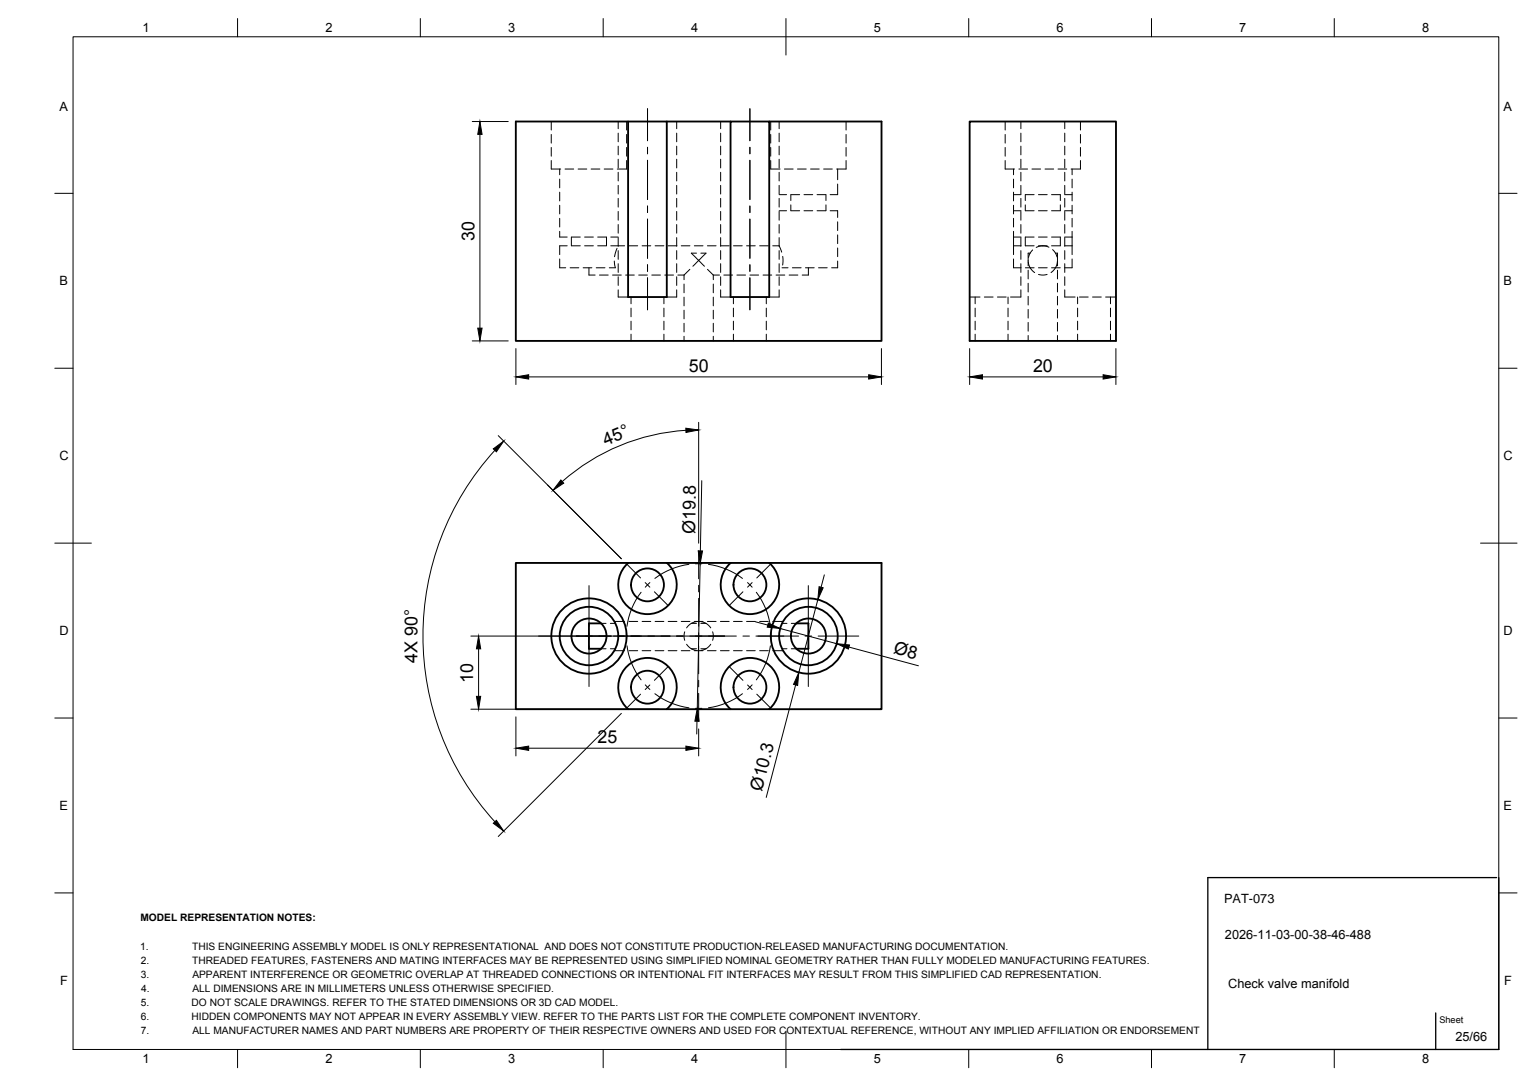
ISO-10303-21;
HEADER;
/* Generated by software containing ST-Developer
 * from STEP Tools, Inc. (www.steptools.com) 
 */

FILE_DESCRIPTION(
/* description */ ('Manual piston pump'),
/* implementation_level */ '2;1');

FILE_NAME(
/* name */ 'Check valve manifold.step',
/* time_stamp */ '2026-11-02T16:54:23-08:00',
/* author */ (''),
/* organization */ (''),
/* preprocessor_version */ 'ST-DEVELOPER v20.2',
/* originating_system */ 'Autodesk Translation Framework v15.17.0.0',
/* authorisation */ '');

FILE_SCHEMA (('AUTOMOTIVE_DESIGN { 1 0 10303 214 3 1 1 }'));
ENDSEC;

DATA;
#10=MECHANICAL_DESIGN_GEOMETRIC_PRESENTATION_REPRESENTATION('',(#725),#19043);
#13=ELLIPSE('',#10933,0.282842712474619,0.2);
#14=ELLIPSE('',#10934,0.282842712474619,0.2);
#15=ELLIPSE('',#10935,0.282842712474619,0.2);
#16=ELLIPSE('',#10936,0.282842712474619,0.2);
#17=ELLIPSE('',#10937,0.282842712474619,0.2);
#18=ELLIPSE('',#10938,0.282842712474619,0.2);
#19=ELLIPSE('',#10939,0.282842712474619,0.2);
#591=SHAPE_REPRESENTATION_RELATIONSHIP('SRR','None',#19338,#654);
#654=ADVANCED_BREP_SHAPE_REPRESENTATION('',(#795),#19005);
#725=STYLED_ITEM('',(#19661),#795);
#795=MANIFOLD_SOLID_BREP('Body1',#9511);
#966=FACE_BOUND('',#2306,.T.);
#967=FACE_BOUND('',#2309,.T.);
#968=FACE_BOUND('',#2312,.T.);
#969=FACE_BOUND('',#2315,.T.);
#970=FACE_BOUND('',#2319,.T.);
#971=FACE_BOUND('',#2320,.T.);
#972=FACE_BOUND('',#2328,.T.);
#973=FACE_BOUND('',#2331,.T.);
#974=FACE_BOUND('',#2336,.T.);
#975=FACE_BOUND('',#2340,.T.);
#976=FACE_BOUND('',#2343,.T.);
#977=FACE_BOUND('',#2348,.T.);
#978=FACE_BOUND('',#2351,.T.);
#979=FACE_BOUND('',#2360,.T.);
#980=FACE_BOUND('',#2361,.T.);
#981=FACE_BOUND('',#2362,.T.);
#982=FACE_BOUND('',#2363,.T.);
#983=FACE_BOUND('',#2364,.T.);
#1069=B_SPLINE_CURVE_WITH_KNOTS('',3,(#16509,#16510,#16511,#16512,#16513,
#16514,#16515,#16516,#16517,#16518,#16519,#16520,#16521,#16522),
 .UNSPECIFIED.,.F.,.F.,(4,2,2,2,2,2,4),(0.307512441683017,0.38428562234823,
0.461058803013443,0.538041843189738,0.615024883366033,0.692007923542328,
0.716698321761712),.UNSPECIFIED.);
#1070=B_SPLINE_CURVE_WITH_KNOTS('',3,(#16524,#16525,#16526,#16527,#16528,
#16529,#16530,#16531,#16532,#16533,#16534,#16535,#16536,#16537,#16538),
 .UNSPECIFIED.,.F.,.F.,(4,2,3,2,2,2,4),(-0.101673438395677,-0.0769830401762948,
0.,0.0769830401762949,0.15396608035259,0.230739261017803,0.307512441683017),
 .UNSPECIFIED.);
#1071=B_SPLINE_CURVE_WITH_KNOTS('',3,(#16573,#16574,#16575,#16576,#16577,
#16578,#16579,#16580,#16581,#16582,#16583,#16584,#16585,#16586),
 .UNSPECIFIED.,.F.,.F.,(4,2,2,2,2,2,4),(-0.716698321761712,-0.692007923542328,
-0.615024883366033,-0.538041843189738,-0.461058803013443,-0.38428562234823,
-0.307512441683017),.UNSPECIFIED.);
#1072=B_SPLINE_CURVE_WITH_KNOTS('',3,(#16590,#16591,#16592,#16593,#16594,
#16595,#16596,#16597,#16598,#16599,#16600,#16601,#16602,#16603,#16604),
 .UNSPECIFIED.,.F.,.F.,(4,2,2,2,3,2,4),(-0.307512441683017,-0.230739261017803,
-0.15396608035259,-0.0769830401762948,0.,0.0769830401762949,0.101673438395681),
 .UNSPECIFIED.);
#1202=CYLINDRICAL_SURFACE('',#10867,0.4);
#1203=CYLINDRICAL_SURFACE('',#10872,0.4);
#1204=CYLINDRICAL_SURFACE('',#10877,0.4);
#1205=CYLINDRICAL_SURFACE('',#10882,0.4);
#1206=CYLINDRICAL_SURFACE('',#10889,0.225);
#1207=CYLINDRICAL_SURFACE('',#10891,0.225);
#1208=CYLINDRICAL_SURFACE('',#10893,0.225);
#1209=CYLINDRICAL_SURFACE('',#10895,0.225);
#1210=CYLINDRICAL_SURFACE('',#10897,0.515);
#1211=CYLINDRICAL_SURFACE('',#10901,0.4);
#1212=CYLINDRICAL_SURFACE('',#10905,0.24);
#1213=CYLINDRICAL_SURFACE('',#10909,0.4);
#1214=CYLINDRICAL_SURFACE('',#10914,0.515);
#1215=CYLINDRICAL_SURFACE('',#10918,0.4);
#1216=CYLINDRICAL_SURFACE('',#10922,0.24);
#1217=CYLINDRICAL_SURFACE('',#10927,0.4);
#1218=CYLINDRICAL_SURFACE('',#10932,0.2);
#1219=CYLINDRICAL_SURFACE('',#10944,0.2);
#1220=CYLINDRICAL_SURFACE('',#10945,0.2);
#1221=CYLINDRICAL_SURFACE('',#10946,0.2);
#1591=FACE_OUTER_BOUND('',#2305,.T.);
#1592=FACE_OUTER_BOUND('',#2307,.T.);
#1593=FACE_OUTER_BOUND('',#2308,.T.);
#1594=FACE_OUTER_BOUND('',#2310,.T.);
#1595=FACE_OUTER_BOUND('',#2311,.T.);
#1596=FACE_OUTER_BOUND('',#2313,.T.);
#1597=FACE_OUTER_BOUND('',#2314,.T.);
#1598=FACE_OUTER_BOUND('',#2316,.T.);
#1599=FACE_OUTER_BOUND('',#2317,.T.);
#1600=FACE_OUTER_BOUND('',#2318,.T.);
#1601=FACE_OUTER_BOUND('',#2321,.T.);
#1602=FACE_OUTER_BOUND('',#2322,.T.);
#1603=FACE_OUTER_BOUND('',#2323,.T.);
#1604=FACE_OUTER_BOUND('',#2324,.T.);
#1605=FACE_OUTER_BOUND('',#2325,.T.);
#1606=FACE_OUTER_BOUND('',#2326,.T.);
#1607=FACE_OUTER_BOUND('',#2327,.T.);
#1608=FACE_OUTER_BOUND('',#2329,.T.);
#1609=FACE_OUTER_BOUND('',#2330,.T.);
#1610=FACE_OUTER_BOUND('',#2332,.T.);
#1611=FACE_OUTER_BOUND('',#2333,.T.);
#1612=FACE_OUTER_BOUND('',#2334,.T.);
#1613=FACE_OUTER_BOUND('',#2335,.T.);
#1614=FACE_OUTER_BOUND('',#2337,.T.);
#1615=FACE_OUTER_BOUND('',#2338,.T.);
#1616=FACE_OUTER_BOUND('',#2339,.T.);
#1617=FACE_OUTER_BOUND('',#2341,.T.);
#1618=FACE_OUTER_BOUND('',#2342,.T.);
#1619=FACE_OUTER_BOUND('',#2344,.T.);
#1620=FACE_OUTER_BOUND('',#2345,.T.);
#1621=FACE_OUTER_BOUND('',#2346,.T.);
#1622=FACE_OUTER_BOUND('',#2347,.T.);
#1623=FACE_OUTER_BOUND('',#2349,.T.);
#1624=FACE_OUTER_BOUND('',#2350,.T.);
#1625=FACE_OUTER_BOUND('',#2352,.T.);
#1626=FACE_OUTER_BOUND('',#2353,.T.);
#1627=FACE_OUTER_BOUND('',#2354,.T.);
#1628=FACE_OUTER_BOUND('',#2355,.T.);
#1629=FACE_OUTER_BOUND('',#2356,.T.);
#1630=FACE_OUTER_BOUND('',#2357,.T.);
#1631=FACE_OUTER_BOUND('',#2358,.T.);
#1632=FACE_OUTER_BOUND('',#2359,.T.);
#2305=EDGE_LOOP('',(#7503,#7504));
#2306=EDGE_LOOP('',(#7505));
#2307=EDGE_LOOP('',(#7506,#7507,#7508,#7509));
#2308=EDGE_LOOP('',(#7510,#7511));
#2309=EDGE_LOOP('',(#7512));
#2310=EDGE_LOOP('',(#7513,#7514,#7515,#7516));
#2311=EDGE_LOOP('',(#7517,#7518));
#2312=EDGE_LOOP('',(#7519));
#2313=EDGE_LOOP('',(#7520,#7521,#7522,#7523));
#2314=EDGE_LOOP('',(#7524,#7525));
#2315=EDGE_LOOP('',(#7526));
#2316=EDGE_LOOP('',(#7527,#7528,#7529,#7530));
#2317=EDGE_LOOP('',(#7531,#7532,#7533,#7534,#7535,#7536,#7537,#7538,#7539,
#7540,#7541,#7542));
#2318=EDGE_LOOP('',(#7543,#7544,#7545,#7546,#7547,#7548,#7549,#7550,#7551,
#7552,#7553,#7554));
#2319=EDGE_LOOP('',(#7555));
#2320=EDGE_LOOP('',(#7556));
#2321=EDGE_LOOP('',(#7557,#7558,#7559,#7560,#7561,#7562,#7563,#7564,#7565,
#7566,#7567,#7568));
#2322=EDGE_LOOP('',(#7569,#7570,#7571,#7572));
#2323=EDGE_LOOP('',(#7573,#7574,#7575,#7576));
#2324=EDGE_LOOP('',(#7577,#7578,#7579,#7580));
#2325=EDGE_LOOP('',(#7581,#7582,#7583,#7584));
#2326=EDGE_LOOP('',(#7585,#7586,#7587,#7588));
#2327=EDGE_LOOP('',(#7589));
#2328=EDGE_LOOP('',(#7590));
#2329=EDGE_LOOP('',(#7591,#7592,#7593,#7594));
#2330=EDGE_LOOP('',(#7595));
#2331=EDGE_LOOP('',(#7596));
#2332=EDGE_LOOP('',(#7597,#7598,#7599,#7600));
#2333=EDGE_LOOP('',(#7601,#7602,#7603,#7604));
#2334=EDGE_LOOP('',(#7605,#7606,#7607,#7608));
#2335=EDGE_LOOP('',(#7609));
#2336=EDGE_LOOP('',(#7610));
#2337=EDGE_LOOP('',(#7611,#7612));
#2338=EDGE_LOOP('',(#7613,#7614,#7615,#7616));
#2339=EDGE_LOOP('',(#7617));
#2340=EDGE_LOOP('',(#7618));
#2341=EDGE_LOOP('',(#7619,#7620,#7621,#7622));
#2342=EDGE_LOOP('',(#7623));
#2343=EDGE_LOOP('',(#7624));
#2344=EDGE_LOOP('',(#7625,#7626,#7627,#7628));
#2345=EDGE_LOOP('',(#7629,#7630,#7631,#7632,#7633));
#2346=EDGE_LOOP('',(#7634,#7635,#7636,#7637,#7638,#7639,#7640));
#2347=EDGE_LOOP('',(#7641));
#2348=EDGE_LOOP('',(#7642));
#2349=EDGE_LOOP('',(#7643,#7644));
#2350=EDGE_LOOP('',(#7645,#7646,#7647,#7648,#7649,#7650,#7651,#7652,#7653,
#7654,#7655,#7656));
#2351=EDGE_LOOP('',(#7657,#7658,#7659,#7660,#7661,#7662,#7663,#7664,#7665));
#2352=EDGE_LOOP('',(#7666,#7667));
#2353=EDGE_LOOP('',(#7668,#7669));
#2354=EDGE_LOOP('',(#7670,#7671,#7672));
#2355=EDGE_LOOP('',(#7673,#7674,#7675));
#2356=EDGE_LOOP('',(#7676,#7677,#7678,#7679,#7680,#7681));
#2357=EDGE_LOOP('',(#7682,#7683,#7684,#7685));
#2358=EDGE_LOOP('',(#7686,#7687,#7688,#7689));
#2359=EDGE_LOOP('',(#7690,#7691,#7692,#7693));
#2360=EDGE_LOOP('',(#7694));
#2361=EDGE_LOOP('',(#7695));
#2362=EDGE_LOOP('',(#7696));
#2363=EDGE_LOOP('',(#7697));
#2364=EDGE_LOOP('',(#7698));
#2947=CIRCLE('',#10865,0.4);
#2948=CIRCLE('',#10866,0.225);
#2949=CIRCLE('',#10868,0.4);
#2950=CIRCLE('',#10870,0.4);
#2951=CIRCLE('',#10871,0.225);
#2952=CIRCLE('',#10873,0.4);
#2953=CIRCLE('',#10875,0.4);
#2954=CIRCLE('',#10876,0.225);
#2955=CIRCLE('',#10878,0.4);
#2956=CIRCLE('',#10880,0.4);
#2957=CIRCLE('',#10881,0.225);
#2958=CIRCLE('',#10883,0.4);
#2959=CIRCLE('',#10886,0.515);
#2960=CIRCLE('',#10887,0.515);
#2961=CIRCLE('',#10890,0.225);
#2962=CIRCLE('',#10892,0.225);
#2963=CIRCLE('',#10894,0.225);
#2964=CIRCLE('',#10896,0.225);
#2965=CIRCLE('',#10898,0.515);
#2966=CIRCLE('',#10900,0.4);
#2967=CIRCLE('',#10902,0.4);
#2968=CIRCLE('',#10904,0.24);
#2969=CIRCLE('',#10906,0.24);
#2970=CIRCLE('',#10908,0.4);
#2971=CIRCLE('',#10910,0.4);
#2972=CIRCLE('',#10913,0.2);
#2973=CIRCLE('',#10915,0.515);
#2974=CIRCLE('',#10917,0.4);
#2975=CIRCLE('',#10919,0.4);
#2976=CIRCLE('',#10921,0.24);
#2977=CIRCLE('',#10923,0.24);
#2978=CIRCLE('',#10925,0.4);
#2979=CIRCLE('',#10926,0.4);
#2980=CIRCLE('',#10928,0.4);
#2981=CIRCLE('',#10931,0.2);
#2982=CIRCLE('',#10941,0.2);
#2983=CIRCLE('',#10943,0.2);
#2984=CIRCLE('',#10947,0.2);
#3445=LINE('',#16386,#4049);
#3446=LINE('',#16392,#4050);
#3447=LINE('',#16395,#4051);
#3448=LINE('',#16399,#4052);
#3449=LINE('',#16405,#4053);
#3450=LINE('',#16408,#4054);
#3451=LINE('',#16412,#4055);
#3452=LINE('',#16418,#4056);
#3453=LINE('',#16421,#4057);
#3454=LINE('',#16425,#4058);
#3455=LINE('',#16431,#4059);
#3456=LINE('',#16434,#4060);
#3457=LINE('',#16436,#4061);
#3458=LINE('',#16438,#4062);
#3459=LINE('',#16440,#4063);
#3460=LINE('',#16442,#4064);
#3461=LINE('',#16444,#4065);
#3462=LINE('',#16445,#4066);
#3463=LINE('',#16448,#4067);
#3464=LINE('',#16449,#4068);
#3465=LINE('',#16450,#4069);
#3466=LINE('',#16452,#4070);
#3467=LINE('',#16453,#4071);
#3468=LINE('',#16460,#4072);
#3469=LINE('',#16462,#4073);
#3470=LINE('',#16463,#4074);
#3471=LINE('',#16467,#4075);
#3472=LINE('',#16471,#4076);
#3473=LINE('',#16475,#4077);
#3474=LINE('',#16479,#4078);
#3475=LINE('',#16483,#4079);
#3476=LINE('',#16490,#4080);
#3477=LINE('',#16497,#4081);
#3478=LINE('',#16501,#4082);
#3479=LINE('',#16505,#4083);
#3480=LINE('',#16506,#4084);
#3481=LINE('',#16545,#4085);
#3482=LINE('',#16552,#4086);
#3483=LINE('',#16559,#4087);
#3484=LINE('',#16563,#4088);
#3485=LINE('',#16569,#4089);
#3486=LINE('',#16570,#4090);
#3487=LINE('',#16588,#4091);
#3488=LINE('',#16609,#4092);
#3489=LINE('',#16616,#4093);
#3490=LINE('',#16623,#4094);
#3491=LINE('',#16635,#4095);
#3492=LINE('',#16637,#4096);
#3493=LINE('',#16639,#4097);
#4049=VECTOR('',#13037,1.);
#4050=VECTOR('',#13044,1.);
#4051=VECTOR('',#13047,1.);
#4052=VECTOR('',#13050,1.);
#4053=VECTOR('',#13057,1.);
#4054=VECTOR('',#13060,1.);
#4055=VECTOR('',#13063,1.);
#4056=VECTOR('',#13070,1.);
#4057=VECTOR('',#13073,1.);
#4058=VECTOR('',#13076,1.);
#4059=VECTOR('',#13083,1.);
#4060=VECTOR('',#13086,1.);
#4061=VECTOR('',#13089,1.);
#4062=VECTOR('',#13090,1.);
#4063=VECTOR('',#13091,1.);
#4064=VECTOR('',#13092,1.);
#4065=VECTOR('',#13093,1.);
#4066=VECTOR('',#13094,1.);
#4067=VECTOR('',#13097,1.);
#4068=VECTOR('',#13098,1.);
#4069=VECTOR('',#13099,1.);
#4070=VECTOR('',#13100,1.);
#4071=VECTOR('',#13101,1.);
#4072=VECTOR('',#13108,1.);
#4073=VECTOR('',#13109,1.);
#4074=VECTOR('',#13110,1.);
#4075=VECTOR('',#13115,0.225);
#4076=VECTOR('',#13120,0.225);
#4077=VECTOR('',#13125,0.225);
#4078=VECTOR('',#13130,0.225);
#4079=VECTOR('',#13135,0.515);
#4080=VECTOR('',#13144,0.4);
#4081=VECTOR('',#13153,0.24);
#4082=VECTOR('',#13156,1.);
#4083=VECTOR('',#13159,1.);
#4084=VECTOR('',#13160,1.);
#4085=VECTOR('',#13175,0.515);
#4086=VECTOR('',#13184,0.4);
#4087=VECTOR('',#13193,0.24);
#4088=VECTOR('',#13196,1.);
#4089=VECTOR('',#13201,1.);
#4090=VECTOR('',#13202,1.);
#4091=VECTOR('',#13205,0.4);
#4092=VECTOR('',#13216,0.2);
#4093=VECTOR('',#13221,1.);
#4094=VECTOR('',#13228,1.);
#4095=VECTOR('',#13249,0.2);
#4096=VECTOR('',#13252,1.);
#4097=VECTOR('',#13255,1.);
#4770=VERTEX_POINT('',#16384);
#4771=VERTEX_POINT('',#16385);
#4772=VERTEX_POINT('',#16388);
#4773=VERTEX_POINT('',#16391);
#4774=VERTEX_POINT('',#16393);
#4775=VERTEX_POINT('',#16397);
#4776=VERTEX_POINT('',#16398);
#4777=VERTEX_POINT('',#16401);
#4778=VERTEX_POINT('',#16404);
#4779=VERTEX_POINT('',#16406);
#4780=VERTEX_POINT('',#16410);
#4781=VERTEX_POINT('',#16411);
#4782=VERTEX_POINT('',#16414);
#4783=VERTEX_POINT('',#16417);
#4784=VERTEX_POINT('',#16419);
#4785=VERTEX_POINT('',#16423);
#4786=VERTEX_POINT('',#16424);
#4787=VERTEX_POINT('',#16427);
#4788=VERTEX_POINT('',#16430);
#4789=VERTEX_POINT('',#16432);
#4790=VERTEX_POINT('',#16437);
#4791=VERTEX_POINT('',#16439);
#4792=VERTEX_POINT('',#16441);
#4793=VERTEX_POINT('',#16443);
#4794=VERTEX_POINT('',#16447);
#4795=VERTEX_POINT('',#16451);
#4796=VERTEX_POINT('',#16454);
#4797=VERTEX_POINT('',#16456);
#4798=VERTEX_POINT('',#16459);
#4799=VERTEX_POINT('',#16461);
#4800=VERTEX_POINT('',#16465);
#4801=VERTEX_POINT('',#16469);
#4802=VERTEX_POINT('',#16473);
#4803=VERTEX_POINT('',#16477);
#4804=VERTEX_POINT('',#16481);
#4805=VERTEX_POINT('',#16485);
#4806=VERTEX_POINT('',#16488);
#4807=VERTEX_POINT('',#16492);
#4808=VERTEX_POINT('',#16495);
#4809=VERTEX_POINT('',#16499);
#4810=VERTEX_POINT('',#16500);
#4811=VERTEX_POINT('',#16502);
#4812=VERTEX_POINT('',#16504);
#4813=VERTEX_POINT('',#16508);
#4814=VERTEX_POINT('',#16543);
#4815=VERTEX_POINT('',#16547);
#4816=VERTEX_POINT('',#16550);
#4817=VERTEX_POINT('',#16554);
#4818=VERTEX_POINT('',#16557);
#4819=VERTEX_POINT('',#16561);
#4820=VERTEX_POINT('',#16562);
#4821=VERTEX_POINT('',#16564);
#4822=VERTEX_POINT('',#16566);
#4823=VERTEX_POINT('',#16568);
#4824=VERTEX_POINT('',#16572);
#4825=VERTEX_POINT('',#16587);
#4826=VERTEX_POINT('',#16610);
#4827=VERTEX_POINT('',#16611);
#4828=VERTEX_POINT('',#16613);
#4829=VERTEX_POINT('',#16615);
#4830=VERTEX_POINT('',#16618);
#4831=VERTEX_POINT('',#16620);
#4832=VERTEX_POINT('',#16622);
#4833=VERTEX_POINT('',#16633);
#5738=EDGE_CURVE('',#4770,#4771,#3445,.T.);
#5739=EDGE_CURVE('',#4770,#4771,#2947,.T.);
#5740=EDGE_CURVE('',#4772,#4772,#2948,.T.);
#5741=EDGE_CURVE('',#4773,#4770,#3446,.T.);
#5742=EDGE_CURVE('',#4774,#4773,#2949,.T.);
#5743=EDGE_CURVE('',#4771,#4774,#3447,.T.);
#5744=EDGE_CURVE('',#4775,#4776,#3448,.T.);
#5745=EDGE_CURVE('',#4775,#4776,#2950,.T.);
#5746=EDGE_CURVE('',#4777,#4777,#2951,.T.);
#5747=EDGE_CURVE('',#4778,#4775,#3449,.T.);
#5748=EDGE_CURVE('',#4779,#4778,#2952,.T.);
#5749=EDGE_CURVE('',#4776,#4779,#3450,.T.);
#5750=EDGE_CURVE('',#4780,#4781,#3451,.T.);
#5751=EDGE_CURVE('',#4780,#4781,#2953,.T.);
#5752=EDGE_CURVE('',#4782,#4782,#2954,.T.);
#5753=EDGE_CURVE('',#4783,#4780,#3452,.T.);
#5754=EDGE_CURVE('',#4784,#4783,#2955,.T.);
#5755=EDGE_CURVE('',#4781,#4784,#3453,.T.);
#5756=EDGE_CURVE('',#4785,#4786,#3454,.T.);
#5757=EDGE_CURVE('',#4785,#4786,#2956,.T.);
#5758=EDGE_CURVE('',#4787,#4787,#2957,.T.);
#5759=EDGE_CURVE('',#4788,#4785,#3455,.T.);
#5760=EDGE_CURVE('',#4789,#4788,#2958,.T.);
#5761=EDGE_CURVE('',#4786,#4789,#3456,.T.);
#5762=EDGE_CURVE('',#4783,#4774,#3457,.T.);
#5763=EDGE_CURVE('',#4790,#4784,#3458,.T.);
#5764=EDGE_CURVE('',#4791,#4790,#3459,.T.);
#5765=EDGE_CURVE('',#4791,#4792,#3460,.T.);
#5766=EDGE_CURVE('',#4792,#4793,#3461,.T.);
#5767=EDGE_CURVE('',#4773,#4793,#3462,.T.);
#5768=EDGE_CURVE('',#4793,#4794,#3463,.T.);
#5769=EDGE_CURVE('',#4794,#4789,#3464,.T.);
#5770=EDGE_CURVE('',#4788,#4779,#3465,.T.);
#5771=EDGE_CURVE('',#4778,#4795,#3466,.T.);
#5772=EDGE_CURVE('',#4795,#4790,#3467,.T.);
#5773=EDGE_CURVE('',#4796,#4796,#2959,.T.);
#5774=EDGE_CURVE('',#4797,#4797,#2960,.T.);
#5775=EDGE_CURVE('',#4798,#4794,#3468,.T.);
#5776=EDGE_CURVE('',#4798,#4799,#3469,.T.);
#5777=EDGE_CURVE('',#4799,#4795,#3470,.T.);
#5778=EDGE_CURVE('',#4800,#4800,#2961,.T.);
#5779=EDGE_CURVE('',#4800,#4772,#3471,.T.);
#5780=EDGE_CURVE('',#4801,#4801,#2962,.T.);
#5781=EDGE_CURVE('',#4801,#4777,#3472,.T.);
#5782=EDGE_CURVE('',#4802,#4802,#2963,.T.);
#5783=EDGE_CURVE('',#4802,#4782,#3473,.T.);
#5784=EDGE_CURVE('',#4803,#4803,#2964,.T.);
#5785=EDGE_CURVE('',#4803,#4787,#3474,.T.);
#5786=EDGE_CURVE('',#4804,#4804,#2965,.T.);
#5787=EDGE_CURVE('',#4804,#4796,#3475,.T.);
#5788=EDGE_CURVE('',#4805,#4805,#2966,.T.);
#5789=EDGE_CURVE('',#4806,#4806,#2967,.T.);
#5790=EDGE_CURVE('',#4806,#4805,#3476,.T.);
#5791=EDGE_CURVE('',#4807,#4807,#2968,.T.);
#5792=EDGE_CURVE('',#4808,#4808,#2969,.T.);
#5793=EDGE_CURVE('',#4808,#4807,#3477,.T.);
#5794=EDGE_CURVE('',#4809,#4810,#3478,.T.);
#5795=EDGE_CURVE('',#4809,#4811,#2970,.T.);
#5796=EDGE_CURVE('',#4812,#4811,#3479,.T.);
#5797=EDGE_CURVE('',#4810,#4812,#3480,.T.);
#5798=EDGE_CURVE('',#4813,#4809,#1069,.T.);
#5799=EDGE_CURVE('',#4813,#4813,#2971,.T.);
#5800=EDGE_CURVE('',#4811,#4813,#1070,.T.);
#5801=EDGE_CURVE('',#4810,#4812,#2972,.T.);
#5802=EDGE_CURVE('',#4814,#4814,#2973,.T.);
#5803=EDGE_CURVE('',#4814,#4797,#3481,.T.);
#5804=EDGE_CURVE('',#4815,#4815,#2974,.T.);
#5805=EDGE_CURVE('',#4816,#4816,#2975,.T.);
#5806=EDGE_CURVE('',#4816,#4815,#3482,.T.);
#5807=EDGE_CURVE('',#4817,#4817,#2976,.T.);
#5808=EDGE_CURVE('',#4818,#4818,#2977,.T.);
#5809=EDGE_CURVE('',#4818,#4817,#3483,.T.);
#5810=EDGE_CURVE('',#4819,#4820,#3484,.T.);
#5811=EDGE_CURVE('',#4819,#4821,#2978,.T.);
#5812=EDGE_CURVE('',#4821,#4822,#2979,.T.);
#5813=EDGE_CURVE('',#4823,#4822,#3485,.T.);
#5814=EDGE_CURVE('',#4820,#4823,#3486,.T.);
#5815=EDGE_CURVE('',#4822,#4824,#1071,.T.);
#5816=EDGE_CURVE('',#4821,#4825,#3487,.T.);
#5817=EDGE_CURVE('',#4825,#4825,#2980,.T.);
#5818=EDGE_CURVE('',#4824,#4819,#1072,.T.);
#5819=EDGE_CURVE('',#4823,#4820,#2981,.T.);
#5820=EDGE_CURVE('',#4824,#4813,#3488,.T.);
#5821=EDGE_CURVE('',#4826,#4827,#13,.T.);
#5822=EDGE_CURVE('',#4828,#4826,#14,.T.);
#5823=EDGE_CURVE('',#4829,#4828,#3489,.T.);
#5824=EDGE_CURVE('',#4826,#4829,#15,.T.);
#5825=EDGE_CURVE('',#4830,#4826,#16,.T.);
#5826=EDGE_CURVE('',#4831,#4830,#17,.T.);
#5827=EDGE_CURVE('',#4832,#4831,#3490,.T.);
#5828=EDGE_CURVE('',#4830,#4832,#18,.T.);
#5829=EDGE_CURVE('',#4827,#4830,#19,.T.);
#5830=EDGE_CURVE('',#4829,#4828,#2982,.T.);
#5831=EDGE_CURVE('',#4832,#4831,#2983,.T.);
#5832=EDGE_CURVE('',#4833,#4833,#2984,.T.);
#5833=EDGE_CURVE('',#4833,#4827,#3491,.T.);
#5834=EDGE_CURVE('',#4792,#4798,#3492,.T.);
#5835=EDGE_CURVE('',#4799,#4791,#3493,.T.);
#7503=ORIENTED_EDGE('',*,*,#5738,.F.);
#7504=ORIENTED_EDGE('',*,*,#5739,.T.);
#7505=ORIENTED_EDGE('',*,*,#5740,.F.);
#7506=ORIENTED_EDGE('',*,*,#5741,.F.);
#7507=ORIENTED_EDGE('',*,*,#5742,.F.);
#7508=ORIENTED_EDGE('',*,*,#5743,.F.);
#7509=ORIENTED_EDGE('',*,*,#5739,.F.);
#7510=ORIENTED_EDGE('',*,*,#5744,.F.);
#7511=ORIENTED_EDGE('',*,*,#5745,.T.);
#7512=ORIENTED_EDGE('',*,*,#5746,.F.);
#7513=ORIENTED_EDGE('',*,*,#5747,.F.);
#7514=ORIENTED_EDGE('',*,*,#5748,.F.);
#7515=ORIENTED_EDGE('',*,*,#5749,.F.);
#7516=ORIENTED_EDGE('',*,*,#5745,.F.);
#7517=ORIENTED_EDGE('',*,*,#5750,.F.);
#7518=ORIENTED_EDGE('',*,*,#5751,.T.);
#7519=ORIENTED_EDGE('',*,*,#5752,.F.);
#7520=ORIENTED_EDGE('',*,*,#5753,.F.);
#7521=ORIENTED_EDGE('',*,*,#5754,.F.);
#7522=ORIENTED_EDGE('',*,*,#5755,.F.);
#7523=ORIENTED_EDGE('',*,*,#5751,.F.);
#7524=ORIENTED_EDGE('',*,*,#5756,.F.);
#7525=ORIENTED_EDGE('',*,*,#5757,.T.);
#7526=ORIENTED_EDGE('',*,*,#5758,.F.);
#7527=ORIENTED_EDGE('',*,*,#5759,.F.);
#7528=ORIENTED_EDGE('',*,*,#5760,.F.);
#7529=ORIENTED_EDGE('',*,*,#5761,.F.);
#7530=ORIENTED_EDGE('',*,*,#5757,.F.);
#7531=ORIENTED_EDGE('',*,*,#5741,.T.);
#7532=ORIENTED_EDGE('',*,*,#5738,.T.);
#7533=ORIENTED_EDGE('',*,*,#5743,.T.);
#7534=ORIENTED_EDGE('',*,*,#5762,.F.);
#7535=ORIENTED_EDGE('',*,*,#5753,.T.);
#7536=ORIENTED_EDGE('',*,*,#5750,.T.);
#7537=ORIENTED_EDGE('',*,*,#5755,.T.);
#7538=ORIENTED_EDGE('',*,*,#5763,.F.);
#7539=ORIENTED_EDGE('',*,*,#5764,.F.);
#7540=ORIENTED_EDGE('',*,*,#5765,.T.);
#7541=ORIENTED_EDGE('',*,*,#5766,.T.);
#7542=ORIENTED_EDGE('',*,*,#5767,.F.);
#7543=ORIENTED_EDGE('',*,*,#5742,.T.);
#7544=ORIENTED_EDGE('',*,*,#5767,.T.);
#7545=ORIENTED_EDGE('',*,*,#5768,.T.);
#7546=ORIENTED_EDGE('',*,*,#5769,.T.);
#7547=ORIENTED_EDGE('',*,*,#5760,.T.);
#7548=ORIENTED_EDGE('',*,*,#5770,.T.);
#7549=ORIENTED_EDGE('',*,*,#5748,.T.);
#7550=ORIENTED_EDGE('',*,*,#5771,.T.);
#7551=ORIENTED_EDGE('',*,*,#5772,.T.);
#7552=ORIENTED_EDGE('',*,*,#5763,.T.);
#7553=ORIENTED_EDGE('',*,*,#5754,.T.);
#7554=ORIENTED_EDGE('',*,*,#5762,.T.);
#7555=ORIENTED_EDGE('',*,*,#5773,.T.);
#7556=ORIENTED_EDGE('',*,*,#5774,.T.);
#7557=ORIENTED_EDGE('',*,*,#5747,.T.);
#7558=ORIENTED_EDGE('',*,*,#5744,.T.);
#7559=ORIENTED_EDGE('',*,*,#5749,.T.);
#7560=ORIENTED_EDGE('',*,*,#5770,.F.);
#7561=ORIENTED_EDGE('',*,*,#5759,.T.);
#7562=ORIENTED_EDGE('',*,*,#5756,.T.);
#7563=ORIENTED_EDGE('',*,*,#5761,.T.);
#7564=ORIENTED_EDGE('',*,*,#5769,.F.);
#7565=ORIENTED_EDGE('',*,*,#5775,.F.);
#7566=ORIENTED_EDGE('',*,*,#5776,.T.);
#7567=ORIENTED_EDGE('',*,*,#5777,.T.);
#7568=ORIENTED_EDGE('',*,*,#5771,.F.);
#7569=ORIENTED_EDGE('',*,*,#5778,.F.);
#7570=ORIENTED_EDGE('',*,*,#5779,.T.);
#7571=ORIENTED_EDGE('',*,*,#5740,.T.);
#7572=ORIENTED_EDGE('',*,*,#5779,.F.);
#7573=ORIENTED_EDGE('',*,*,#5780,.F.);
#7574=ORIENTED_EDGE('',*,*,#5781,.T.);
#7575=ORIENTED_EDGE('',*,*,#5746,.T.);
#7576=ORIENTED_EDGE('',*,*,#5781,.F.);
#7577=ORIENTED_EDGE('',*,*,#5782,.F.);
#7578=ORIENTED_EDGE('',*,*,#5783,.T.);
#7579=ORIENTED_EDGE('',*,*,#5752,.T.);
#7580=ORIENTED_EDGE('',*,*,#5783,.F.);
#7581=ORIENTED_EDGE('',*,*,#5784,.F.);
#7582=ORIENTED_EDGE('',*,*,#5785,.T.);
#7583=ORIENTED_EDGE('',*,*,#5758,.T.);
#7584=ORIENTED_EDGE('',*,*,#5785,.F.);
#7585=ORIENTED_EDGE('',*,*,#5786,.F.);
#7586=ORIENTED_EDGE('',*,*,#5787,.T.);
#7587=ORIENTED_EDGE('',*,*,#5773,.F.);
#7588=ORIENTED_EDGE('',*,*,#5787,.F.);
#7589=ORIENTED_EDGE('',*,*,#5786,.T.);
#7590=ORIENTED_EDGE('',*,*,#5788,.F.);
#7591=ORIENTED_EDGE('',*,*,#5789,.F.);
#7592=ORIENTED_EDGE('',*,*,#5790,.T.);
#7593=ORIENTED_EDGE('',*,*,#5788,.T.);
#7594=ORIENTED_EDGE('',*,*,#5790,.F.);
#7595=ORIENTED_EDGE('',*,*,#5789,.T.);
#7596=ORIENTED_EDGE('',*,*,#5791,.F.);
#7597=ORIENTED_EDGE('',*,*,#5792,.F.);
#7598=ORIENTED_EDGE('',*,*,#5793,.T.);
#7599=ORIENTED_EDGE('',*,*,#5791,.T.);
#7600=ORIENTED_EDGE('',*,*,#5793,.F.);
#7601=ORIENTED_EDGE('',*,*,#5794,.F.);
#7602=ORIENTED_EDGE('',*,*,#5795,.T.);
#7603=ORIENTED_EDGE('',*,*,#5796,.F.);
#7604=ORIENTED_EDGE('',*,*,#5797,.F.);
#7605=ORIENTED_EDGE('',*,*,#5798,.F.);
#7606=ORIENTED_EDGE('',*,*,#5799,.T.);
#7607=ORIENTED_EDGE('',*,*,#5800,.F.);
#7608=ORIENTED_EDGE('',*,*,#5795,.F.);
#7609=ORIENTED_EDGE('',*,*,#5799,.F.);
#7610=ORIENTED_EDGE('',*,*,#5792,.T.);
#7611=ORIENTED_EDGE('',*,*,#5797,.T.);
#7612=ORIENTED_EDGE('',*,*,#5801,.F.);
#7613=ORIENTED_EDGE('',*,*,#5802,.F.);
#7614=ORIENTED_EDGE('',*,*,#5803,.T.);
#7615=ORIENTED_EDGE('',*,*,#5774,.F.);
#7616=ORIENTED_EDGE('',*,*,#5803,.F.);
#7617=ORIENTED_EDGE('',*,*,#5802,.T.);
#7618=ORIENTED_EDGE('',*,*,#5804,.F.);
#7619=ORIENTED_EDGE('',*,*,#5805,.F.);
#7620=ORIENTED_EDGE('',*,*,#5806,.T.);
#7621=ORIENTED_EDGE('',*,*,#5804,.T.);
#7622=ORIENTED_EDGE('',*,*,#5806,.F.);
#7623=ORIENTED_EDGE('',*,*,#5805,.T.);
#7624=ORIENTED_EDGE('',*,*,#5807,.F.);
#7625=ORIENTED_EDGE('',*,*,#5808,.F.);
#7626=ORIENTED_EDGE('',*,*,#5809,.T.);
#7627=ORIENTED_EDGE('',*,*,#5807,.T.);
#7628=ORIENTED_EDGE('',*,*,#5809,.F.);
#7629=ORIENTED_EDGE('',*,*,#5810,.F.);
#7630=ORIENTED_EDGE('',*,*,#5811,.T.);
#7631=ORIENTED_EDGE('',*,*,#5812,.T.);
#7632=ORIENTED_EDGE('',*,*,#5813,.F.);
#7633=ORIENTED_EDGE('',*,*,#5814,.F.);
#7634=ORIENTED_EDGE('',*,*,#5815,.F.);
#7635=ORIENTED_EDGE('',*,*,#5812,.F.);
#7636=ORIENTED_EDGE('',*,*,#5816,.T.);
#7637=ORIENTED_EDGE('',*,*,#5817,.T.);
#7638=ORIENTED_EDGE('',*,*,#5816,.F.);
#7639=ORIENTED_EDGE('',*,*,#5811,.F.);
#7640=ORIENTED_EDGE('',*,*,#5818,.F.);
#7641=ORIENTED_EDGE('',*,*,#5817,.F.);
#7642=ORIENTED_EDGE('',*,*,#5808,.T.);
#7643=ORIENTED_EDGE('',*,*,#5814,.T.);
#7644=ORIENTED_EDGE('',*,*,#5819,.T.);
#7645=ORIENTED_EDGE('',*,*,#5810,.T.);
#7646=ORIENTED_EDGE('',*,*,#5819,.F.);
#7647=ORIENTED_EDGE('',*,*,#5813,.T.);
#7648=ORIENTED_EDGE('',*,*,#5815,.T.);
#7649=ORIENTED_EDGE('',*,*,#5820,.T.);
#7650=ORIENTED_EDGE('',*,*,#5798,.T.);
#7651=ORIENTED_EDGE('',*,*,#5794,.T.);
#7652=ORIENTED_EDGE('',*,*,#5801,.T.);
#7653=ORIENTED_EDGE('',*,*,#5796,.T.);
#7654=ORIENTED_EDGE('',*,*,#5800,.T.);
#7655=ORIENTED_EDGE('',*,*,#5820,.F.);
#7656=ORIENTED_EDGE('',*,*,#5818,.T.);
#7657=ORIENTED_EDGE('',*,*,#5821,.F.);
#7658=ORIENTED_EDGE('',*,*,#5822,.F.);
#7659=ORIENTED_EDGE('',*,*,#5823,.F.);
#7660=ORIENTED_EDGE('',*,*,#5824,.F.);
#7661=ORIENTED_EDGE('',*,*,#5825,.F.);
#7662=ORIENTED_EDGE('',*,*,#5826,.F.);
#7663=ORIENTED_EDGE('',*,*,#5827,.F.);
#7664=ORIENTED_EDGE('',*,*,#5828,.F.);
#7665=ORIENTED_EDGE('',*,*,#5829,.F.);
#7666=ORIENTED_EDGE('',*,*,#5823,.T.);
#7667=ORIENTED_EDGE('',*,*,#5830,.F.);
#7668=ORIENTED_EDGE('',*,*,#5827,.T.);
#7669=ORIENTED_EDGE('',*,*,#5831,.F.);
#7670=ORIENTED_EDGE('',*,*,#5822,.T.);
#7671=ORIENTED_EDGE('',*,*,#5824,.T.);
#7672=ORIENTED_EDGE('',*,*,#5830,.T.);
#7673=ORIENTED_EDGE('',*,*,#5828,.T.);
#7674=ORIENTED_EDGE('',*,*,#5831,.T.);
#7675=ORIENTED_EDGE('',*,*,#5826,.T.);
#7676=ORIENTED_EDGE('',*,*,#5832,.F.);
#7677=ORIENTED_EDGE('',*,*,#5833,.T.);
#7678=ORIENTED_EDGE('',*,*,#5829,.T.);
#7679=ORIENTED_EDGE('',*,*,#5825,.T.);
#7680=ORIENTED_EDGE('',*,*,#5821,.T.);
#7681=ORIENTED_EDGE('',*,*,#5833,.F.);
#7682=ORIENTED_EDGE('',*,*,#5834,.T.);
#7683=ORIENTED_EDGE('',*,*,#5775,.T.);
#7684=ORIENTED_EDGE('',*,*,#5768,.F.);
#7685=ORIENTED_EDGE('',*,*,#5766,.F.);
#7686=ORIENTED_EDGE('',*,*,#5835,.T.);
#7687=ORIENTED_EDGE('',*,*,#5764,.T.);
#7688=ORIENTED_EDGE('',*,*,#5772,.F.);
#7689=ORIENTED_EDGE('',*,*,#5777,.F.);
#7690=ORIENTED_EDGE('',*,*,#5835,.F.);
#7691=ORIENTED_EDGE('',*,*,#5776,.F.);
#7692=ORIENTED_EDGE('',*,*,#5834,.F.);
#7693=ORIENTED_EDGE('',*,*,#5765,.F.);
#7694=ORIENTED_EDGE('',*,*,#5832,.T.);
#7695=ORIENTED_EDGE('',*,*,#5784,.T.);
#7696=ORIENTED_EDGE('',*,*,#5782,.T.);
#7697=ORIENTED_EDGE('',*,*,#5780,.T.);
#7698=ORIENTED_EDGE('',*,*,#5778,.T.);
#8728=PLANE('',#10864);
#8729=PLANE('',#10869);
#8730=PLANE('',#10874);
#8731=PLANE('',#10879);
#8732=PLANE('',#10884);
#8733=PLANE('',#10885);
#8734=PLANE('',#10888);
#8735=PLANE('',#10899);
#8736=PLANE('',#10903);
#8737=PLANE('',#10907);
#8738=PLANE('',#10911);
#8739=PLANE('',#10912);
#8740=PLANE('',#10916);
#8741=PLANE('',#10920);
#8742=PLANE('',#10924);
#8743=PLANE('',#10929);
#8744=PLANE('',#10930);
#8745=PLANE('',#10940);
#8746=PLANE('',#10942);
#8747=PLANE('',#10948);
#8748=PLANE('',#10949);
#8749=PLANE('',#10950);
#9196=ADVANCED_FACE('',(#1591,#966),#8728,.T.);
#9197=ADVANCED_FACE('',(#1592),#1202,.F.);
#9198=ADVANCED_FACE('',(#1593,#967),#8729,.T.);
#9199=ADVANCED_FACE('',(#1594),#1203,.F.);
#9200=ADVANCED_FACE('',(#1595,#968),#8730,.T.);
#9201=ADVANCED_FACE('',(#1596),#1204,.F.);
#9202=ADVANCED_FACE('',(#1597,#969),#8731,.T.);
#9203=ADVANCED_FACE('',(#1598),#1205,.F.);
#9204=ADVANCED_FACE('',(#1599),#8732,.T.);
#9205=ADVANCED_FACE('',(#1600,#970,#971),#8733,.T.);
#9206=ADVANCED_FACE('',(#1601),#8734,.T.);
#9207=ADVANCED_FACE('',(#1602),#1206,.F.);
#9208=ADVANCED_FACE('',(#1603),#1207,.F.);
#9209=ADVANCED_FACE('',(#1604),#1208,.F.);
#9210=ADVANCED_FACE('',(#1605),#1209,.F.);
#9211=ADVANCED_FACE('',(#1606),#1210,.F.);
#9212=ADVANCED_FACE('',(#1607,#972),#8735,.T.);
#9213=ADVANCED_FACE('',(#1608),#1211,.F.);
#9214=ADVANCED_FACE('',(#1609,#973),#8736,.T.);
#9215=ADVANCED_FACE('',(#1610),#1212,.F.);
#9216=ADVANCED_FACE('',(#1611),#8737,.T.);
#9217=ADVANCED_FACE('',(#1612),#1213,.F.);
#9218=ADVANCED_FACE('',(#1613,#974),#8738,.F.);
#9219=ADVANCED_FACE('',(#1614),#8739,.F.);
#9220=ADVANCED_FACE('',(#1615),#1214,.F.);
#9221=ADVANCED_FACE('',(#1616,#975),#8740,.T.);
#9222=ADVANCED_FACE('',(#1617),#1215,.F.);
#9223=ADVANCED_FACE('',(#1618,#976),#8741,.T.);
#9224=ADVANCED_FACE('',(#1619),#1216,.F.);
#9225=ADVANCED_FACE('',(#1620),#8742,.T.);
#9226=ADVANCED_FACE('',(#1621),#1217,.F.);
#9227=ADVANCED_FACE('',(#1622,#977),#8743,.F.);
#9228=ADVANCED_FACE('',(#1623),#8744,.T.);
#9229=ADVANCED_FACE('',(#1624,#978),#1218,.F.);
#9230=ADVANCED_FACE('',(#1625),#8745,.F.);
#9231=ADVANCED_FACE('',(#1626),#8746,.F.);
#9232=ADVANCED_FACE('',(#1627),#1219,.F.);
#9233=ADVANCED_FACE('',(#1628),#1220,.F.);
#9234=ADVANCED_FACE('',(#1629),#1221,.F.);
#9235=ADVANCED_FACE('',(#1630),#8747,.T.);
#9236=ADVANCED_FACE('',(#1631),#8748,.T.);
#9237=ADVANCED_FACE('',(#1632,#979,#980,#981,#982,#983),#8749,.F.);
#9511=CLOSED_SHELL('',(#9196,#9197,#9198,#9199,#9200,#9201,#9202,#9203,
#9204,#9205,#9206,#9207,#9208,#9209,#9210,#9211,#9212,#9213,#9214,#9215,
#9216,#9217,#9218,#9219,#9220,#9221,#9222,#9223,#9224,#9225,#9226,#9227,
#9228,#9229,#9230,#9231,#9232,#9233,#9234,#9235,#9236,#9237));
#10863=AXIS2_PLACEMENT_3D('',#16382,#13033,#13034);
#10864=AXIS2_PLACEMENT_3D('',#16383,#13035,#13036);
#10865=AXIS2_PLACEMENT_3D('',#16387,#13038,#13039);
#10866=AXIS2_PLACEMENT_3D('',#16389,#13040,#13041);
#10867=AXIS2_PLACEMENT_3D('',#16390,#13042,#13043);
#10868=AXIS2_PLACEMENT_3D('',#16394,#13045,#13046);
#10869=AXIS2_PLACEMENT_3D('',#16396,#13048,#13049);
#10870=AXIS2_PLACEMENT_3D('',#16400,#13051,#13052);
#10871=AXIS2_PLACEMENT_3D('',#16402,#13053,#13054);
#10872=AXIS2_PLACEMENT_3D('',#16403,#13055,#13056);
#10873=AXIS2_PLACEMENT_3D('',#16407,#13058,#13059);
#10874=AXIS2_PLACEMENT_3D('',#16409,#13061,#13062);
#10875=AXIS2_PLACEMENT_3D('',#16413,#13064,#13065);
#10876=AXIS2_PLACEMENT_3D('',#16415,#13066,#13067);
#10877=AXIS2_PLACEMENT_3D('',#16416,#13068,#13069);
#10878=AXIS2_PLACEMENT_3D('',#16420,#13071,#13072);
#10879=AXIS2_PLACEMENT_3D('',#16422,#13074,#13075);
#10880=AXIS2_PLACEMENT_3D('',#16426,#13077,#13078);
#10881=AXIS2_PLACEMENT_3D('',#16428,#13079,#13080);
#10882=AXIS2_PLACEMENT_3D('',#16429,#13081,#13082);
#10883=AXIS2_PLACEMENT_3D('',#16433,#13084,#13085);
#10884=AXIS2_PLACEMENT_3D('',#16435,#13087,#13088);
#10885=AXIS2_PLACEMENT_3D('',#16446,#13095,#13096);
#10886=AXIS2_PLACEMENT_3D('',#16455,#13102,#13103);
#10887=AXIS2_PLACEMENT_3D('',#16457,#13104,#13105);
#10888=AXIS2_PLACEMENT_3D('',#16458,#13106,#13107);
#10889=AXIS2_PLACEMENT_3D('',#16464,#13111,#13112);
#10890=AXIS2_PLACEMENT_3D('',#16466,#13113,#13114);
#10891=AXIS2_PLACEMENT_3D('',#16468,#13116,#13117);
#10892=AXIS2_PLACEMENT_3D('',#16470,#13118,#13119);
#10893=AXIS2_PLACEMENT_3D('',#16472,#13121,#13122);
#10894=AXIS2_PLACEMENT_3D('',#16474,#13123,#13124);
#10895=AXIS2_PLACEMENT_3D('',#16476,#13126,#13127);
#10896=AXIS2_PLACEMENT_3D('',#16478,#13128,#13129);
#10897=AXIS2_PLACEMENT_3D('',#16480,#13131,#13132);
#10898=AXIS2_PLACEMENT_3D('',#16482,#13133,#13134);
#10899=AXIS2_PLACEMENT_3D('',#16484,#13136,#13137);
#10900=AXIS2_PLACEMENT_3D('',#16486,#13138,#13139);
#10901=AXIS2_PLACEMENT_3D('',#16487,#13140,#13141);
#10902=AXIS2_PLACEMENT_3D('',#16489,#13142,#13143);
#10903=AXIS2_PLACEMENT_3D('',#16491,#13145,#13146);
#10904=AXIS2_PLACEMENT_3D('',#16493,#13147,#13148);
#10905=AXIS2_PLACEMENT_3D('',#16494,#13149,#13150);
#10906=AXIS2_PLACEMENT_3D('',#16496,#13151,#13152);
#10907=AXIS2_PLACEMENT_3D('',#16498,#13154,#13155);
#10908=AXIS2_PLACEMENT_3D('',#16503,#13157,#13158);
#10909=AXIS2_PLACEMENT_3D('',#16507,#13161,#13162);
#10910=AXIS2_PLACEMENT_3D('',#16523,#13163,#13164);
#10911=AXIS2_PLACEMENT_3D('',#16539,#13165,#13166);
#10912=AXIS2_PLACEMENT_3D('',#16540,#13167,#13168);
#10913=AXIS2_PLACEMENT_3D('',#16541,#13169,#13170);
#10914=AXIS2_PLACEMENT_3D('',#16542,#13171,#13172);
#10915=AXIS2_PLACEMENT_3D('',#16544,#13173,#13174);
#10916=AXIS2_PLACEMENT_3D('',#16546,#13176,#13177);
#10917=AXIS2_PLACEMENT_3D('',#16548,#13178,#13179);
#10918=AXIS2_PLACEMENT_3D('',#16549,#13180,#13181);
#10919=AXIS2_PLACEMENT_3D('',#16551,#13182,#13183);
#10920=AXIS2_PLACEMENT_3D('',#16553,#13185,#13186);
#10921=AXIS2_PLACEMENT_3D('',#16555,#13187,#13188);
#10922=AXIS2_PLACEMENT_3D('',#16556,#13189,#13190);
#10923=AXIS2_PLACEMENT_3D('',#16558,#13191,#13192);
#10924=AXIS2_PLACEMENT_3D('',#16560,#13194,#13195);
#10925=AXIS2_PLACEMENT_3D('',#16565,#13197,#13198);
#10926=AXIS2_PLACEMENT_3D('',#16567,#13199,#13200);
#10927=AXIS2_PLACEMENT_3D('',#16571,#13203,#13204);
#10928=AXIS2_PLACEMENT_3D('',#16589,#13206,#13207);
#10929=AXIS2_PLACEMENT_3D('',#16605,#13208,#13209);
#10930=AXIS2_PLACEMENT_3D('',#16606,#13210,#13211);
#10931=AXIS2_PLACEMENT_3D('',#16607,#13212,#13213);
#10932=AXIS2_PLACEMENT_3D('',#16608,#13214,#13215);
#10933=AXIS2_PLACEMENT_3D('',#16612,#13217,#13218);
#10934=AXIS2_PLACEMENT_3D('',#16614,#13219,#13220);
#10935=AXIS2_PLACEMENT_3D('',#16617,#13222,#13223);
#10936=AXIS2_PLACEMENT_3D('',#16619,#13224,#13225);
#10937=AXIS2_PLACEMENT_3D('',#16621,#13226,#13227);
#10938=AXIS2_PLACEMENT_3D('',#16624,#13229,#13230);
#10939=AXIS2_PLACEMENT_3D('',#16625,#13231,#13232);
#10940=AXIS2_PLACEMENT_3D('',#16626,#13233,#13234);
#10941=AXIS2_PLACEMENT_3D('',#16627,#13235,#13236);
#10942=AXIS2_PLACEMENT_3D('',#16628,#13237,#13238);
#10943=AXIS2_PLACEMENT_3D('',#16629,#13239,#13240);
#10944=AXIS2_PLACEMENT_3D('',#16630,#13241,#13242);
#10945=AXIS2_PLACEMENT_3D('',#16631,#13243,#13244);
#10946=AXIS2_PLACEMENT_3D('',#16632,#13245,#13246);
#10947=AXIS2_PLACEMENT_3D('',#16634,#13247,#13248);
#10948=AXIS2_PLACEMENT_3D('',#16636,#13250,#13251);
#10949=AXIS2_PLACEMENT_3D('',#16638,#13253,#13254);
#10950=AXIS2_PLACEMENT_3D('',#16640,#13256,#13257);
#13033=DIRECTION('axis',(0.,0.,1.));
#13034=DIRECTION('refdir',(1.,0.,0.));
#13035=DIRECTION('center_axis',(0.,0.,1.));
#13036=DIRECTION('ref_axis',(1.,0.,0.));
#13037=DIRECTION('',(-1.,0.,0.));
#13038=DIRECTION('center_axis',(0.,0.,1.));
#13039=DIRECTION('ref_axis',(1.,0.,0.));
#13040=DIRECTION('center_axis',(0.,0.,1.));
#13041=DIRECTION('ref_axis',(1.,0.,0.));
#13042=DIRECTION('center_axis',(0.,0.,1.));
#13043=DIRECTION('ref_axis',(6.12323399573677E-17,1.,0.));
#13044=DIRECTION('',(0.,0.,-1.));
#13045=DIRECTION('center_axis',(0.,0.,-1.));
#13046=DIRECTION('ref_axis',(1.,0.,0.));
#13047=DIRECTION('',(0.,0.,1.));
#13048=DIRECTION('center_axis',(0.,0.,1.));
#13049=DIRECTION('ref_axis',(1.,0.,0.));
#13050=DIRECTION('',(1.,0.,0.));
#13051=DIRECTION('center_axis',(0.,0.,1.));
#13052=DIRECTION('ref_axis',(1.,0.,0.));
#13053=DIRECTION('center_axis',(0.,0.,1.));
#13054=DIRECTION('ref_axis',(1.,0.,0.));
#13055=DIRECTION('center_axis',(0.,0.,1.));
#13056=DIRECTION('ref_axis',(-1.83697019872103E-16,-1.,0.));
#13057=DIRECTION('',(0.,0.,-1.));
#13058=DIRECTION('center_axis',(0.,0.,-1.));
#13059=DIRECTION('ref_axis',(1.,0.,0.));
#13060=DIRECTION('',(0.,0.,1.));
#13061=DIRECTION('center_axis',(0.,0.,1.));
#13062=DIRECTION('ref_axis',(1.,0.,0.));
#13063=DIRECTION('',(-1.,0.,0.));
#13064=DIRECTION('center_axis',(0.,0.,1.));
#13065=DIRECTION('ref_axis',(1.,0.,0.));
#13066=DIRECTION('center_axis',(0.,0.,1.));
#13067=DIRECTION('ref_axis',(1.,0.,0.));
#13068=DIRECTION('center_axis',(0.,0.,1.));
#13069=DIRECTION('ref_axis',(2.83276944882399E-16,1.,0.));
#13070=DIRECTION('',(0.,0.,-1.));
#13071=DIRECTION('center_axis',(0.,0.,-1.));
#13072=DIRECTION('ref_axis',(1.,0.,0.));
#13073=DIRECTION('',(0.,0.,1.));
#13074=DIRECTION('center_axis',(0.,0.,1.));
#13075=DIRECTION('ref_axis',(1.,0.,0.));
#13076=DIRECTION('',(1.,0.,0.));
#13077=DIRECTION('center_axis',(0.,0.,1.));
#13078=DIRECTION('ref_axis',(1.,0.,0.));
#13079=DIRECTION('center_axis',(0.,0.,1.));
#13080=DIRECTION('ref_axis',(1.,0.,0.));
#13081=DIRECTION('center_axis',(0.,0.,1.));
#13082=DIRECTION('ref_axis',(-1.83697019872103E-16,-1.,0.));
#13083=DIRECTION('',(0.,0.,-1.));
#13084=DIRECTION('center_axis',(0.,0.,-1.));
#13085=DIRECTION('ref_axis',(1.,0.,0.));
#13086=DIRECTION('',(0.,0.,1.));
#13087=DIRECTION('center_axis',(0.,-1.,0.));
#13088=DIRECTION('ref_axis',(1.,0.,0.));
#13089=DIRECTION('',(1.,0.,0.));
#13090=DIRECTION('',(1.,0.,0.));
#13091=DIRECTION('',(0.,0.,1.));
#13092=DIRECTION('',(1.,0.,0.));
#13093=DIRECTION('',(0.,0.,1.));
#13094=DIRECTION('',(1.,0.,0.));
#13095=DIRECTION('center_axis',(0.,0.,1.));
#13096=DIRECTION('ref_axis',(1.,0.,0.));
#13097=DIRECTION('',(0.,1.,0.));
#13098=DIRECTION('',(-1.,0.,0.));
#13099=DIRECTION('',(-1.,0.,0.));
#13100=DIRECTION('',(-1.,0.,0.));
#13101=DIRECTION('',(0.,-1.,0.));
#13102=DIRECTION('center_axis',(0.,0.,-1.));
#13103=DIRECTION('ref_axis',(1.,0.,0.));
#13104=DIRECTION('center_axis',(0.,0.,-1.));
#13105=DIRECTION('ref_axis',(1.,0.,0.));
#13106=DIRECTION('center_axis',(0.,1.,0.));
#13107=DIRECTION('ref_axis',(-1.,0.,0.));
#13108=DIRECTION('',(0.,0.,1.));
#13109=DIRECTION('',(-1.,0.,0.));
#13110=DIRECTION('',(0.,0.,1.));
#13111=DIRECTION('center_axis',(0.,0.,1.));
#13112=DIRECTION('ref_axis',(1.,0.,0.));
#13113=DIRECTION('center_axis',(0.,0.,1.));
#13114=DIRECTION('ref_axis',(1.,0.,0.));
#13115=DIRECTION('',(0.,0.,1.));
#13116=DIRECTION('center_axis',(0.,0.,1.));
#13117=DIRECTION('ref_axis',(1.,0.,0.));
#13118=DIRECTION('center_axis',(0.,0.,1.));
#13119=DIRECTION('ref_axis',(1.,0.,0.));
#13120=DIRECTION('',(0.,0.,1.));
#13121=DIRECTION('center_axis',(0.,0.,1.));
#13122=DIRECTION('ref_axis',(1.,0.,0.));
#13123=DIRECTION('center_axis',(0.,0.,1.));
#13124=DIRECTION('ref_axis',(1.,0.,0.));
#13125=DIRECTION('',(0.,0.,1.));
#13126=DIRECTION('center_axis',(0.,0.,1.));
#13127=DIRECTION('ref_axis',(1.,0.,0.));
#13128=DIRECTION('center_axis',(0.,0.,1.));
#13129=DIRECTION('ref_axis',(1.,0.,0.));
#13130=DIRECTION('',(0.,0.,1.));
#13131=DIRECTION('center_axis',(0.,0.,1.));
#13132=DIRECTION('ref_axis',(1.,0.,0.));
#13133=DIRECTION('center_axis',(0.,0.,1.));
#13134=DIRECTION('ref_axis',(1.,0.,0.));
#13135=DIRECTION('',(0.,0.,1.));
#13136=DIRECTION('center_axis',(0.,0.,1.));
#13137=DIRECTION('ref_axis',(1.,0.,0.));
#13138=DIRECTION('center_axis',(0.,0.,1.));
#13139=DIRECTION('ref_axis',(1.,0.,0.));
#13140=DIRECTION('center_axis',(0.,0.,1.));
#13141=DIRECTION('ref_axis',(1.,0.,0.));
#13142=DIRECTION('center_axis',(0.,0.,1.));
#13143=DIRECTION('ref_axis',(1.,0.,0.));
#13144=DIRECTION('',(0.,0.,1.));
#13145=DIRECTION('center_axis',(0.,0.,1.));
#13146=DIRECTION('ref_axis',(1.,0.,0.));
#13147=DIRECTION('center_axis',(0.,0.,1.));
#13148=DIRECTION('ref_axis',(1.,0.,0.));
#13149=DIRECTION('center_axis',(0.,0.,1.));
#13150=DIRECTION('ref_axis',(1.,0.,0.));
#13151=DIRECTION('center_axis',(0.,0.,1.));
#13152=DIRECTION('ref_axis',(1.,0.,0.));
#13153=DIRECTION('',(0.,0.,1.));
#13154=DIRECTION('center_axis',(0.,0.,1.));
#13155=DIRECTION('ref_axis',(1.,0.,0.));
#13156=DIRECTION('',(1.,0.,0.));
#13157=DIRECTION('center_axis',(0.,0.,1.));
#13158=DIRECTION('ref_axis',(1.,0.,0.));
#13159=DIRECTION('',(-1.,0.,0.));
#13160=DIRECTION('',(0.,1.,0.));
#13161=DIRECTION('center_axis',(0.,0.,1.));
#13162=DIRECTION('ref_axis',(1.,0.,0.));
#13163=DIRECTION('center_axis',(0.,0.,1.));
#13164=DIRECTION('ref_axis',(1.,0.,0.));
#13165=DIRECTION('center_axis',(0.,0.,1.));
#13166=DIRECTION('ref_axis',(1.,0.,0.));
#13167=DIRECTION('center_axis',(1.,0.,0.));
#13168=DIRECTION('ref_axis',(0.,0.,-1.));
#13169=DIRECTION('center_axis',(1.,0.,0.));
#13170=DIRECTION('ref_axis',(0.,0.,-1.));
#13171=DIRECTION('center_axis',(0.,0.,1.));
#13172=DIRECTION('ref_axis',(1.,0.,0.));
#13173=DIRECTION('center_axis',(0.,0.,1.));
#13174=DIRECTION('ref_axis',(1.,0.,0.));
#13175=DIRECTION('',(0.,0.,1.));
#13176=DIRECTION('center_axis',(0.,0.,1.));
#13177=DIRECTION('ref_axis',(1.,0.,0.));
#13178=DIRECTION('center_axis',(0.,0.,1.));
#13179=DIRECTION('ref_axis',(1.,0.,0.));
#13180=DIRECTION('center_axis',(0.,0.,1.));
#13181=DIRECTION('ref_axis',(1.,0.,0.));
#13182=DIRECTION('center_axis',(0.,0.,1.));
#13183=DIRECTION('ref_axis',(1.,0.,0.));
#13184=DIRECTION('',(0.,0.,1.));
#13185=DIRECTION('center_axis',(0.,0.,1.));
#13186=DIRECTION('ref_axis',(1.,0.,0.));
#13187=DIRECTION('center_axis',(0.,0.,1.));
#13188=DIRECTION('ref_axis',(1.,0.,0.));
#13189=DIRECTION('center_axis',(0.,0.,1.));
#13190=DIRECTION('ref_axis',(1.,0.,0.));
#13191=DIRECTION('center_axis',(0.,0.,1.));
#13192=DIRECTION('ref_axis',(1.,0.,0.));
#13193=DIRECTION('',(0.,0.,1.));
#13194=DIRECTION('center_axis',(0.,0.,1.));
#13195=DIRECTION('ref_axis',(1.,0.,0.));
#13196=DIRECTION('',(-1.,0.,0.));
#13197=DIRECTION('center_axis',(0.,0.,1.));
#13198=DIRECTION('ref_axis',(1.,0.,0.));
#13199=DIRECTION('center_axis',(0.,0.,1.));
#13200=DIRECTION('ref_axis',(1.,0.,0.));
#13201=DIRECTION('',(1.,0.,0.));
#13202=DIRECTION('',(0.,-1.,0.));
#13203=DIRECTION('center_axis',(0.,0.,1.));
#13204=DIRECTION('ref_axis',(1.,0.,0.));
#13205=DIRECTION('',(0.,0.,1.));
#13206=DIRECTION('center_axis',(0.,0.,1.));
#13207=DIRECTION('ref_axis',(1.,0.,0.));
#13208=DIRECTION('center_axis',(0.,0.,1.));
#13209=DIRECTION('ref_axis',(1.,0.,0.));
#13210=DIRECTION('center_axis',(1.,0.,0.));
#13211=DIRECTION('ref_axis',(0.,0.,-1.));
#13212=DIRECTION('center_axis',(1.,0.,0.));
#13213=DIRECTION('ref_axis',(0.,0.,-1.));
#13214=DIRECTION('center_axis',(1.,0.,0.));
#13215=DIRECTION('ref_axis',(0.,0.,-1.));
#13216=DIRECTION('',(1.,0.,0.));
#13217=DIRECTION('center_axis',(-0.707106781186549,0.,0.707106781186546));
#13218=DIRECTION('ref_axis',(-0.707106781186546,0.,-0.707106781186549));
#13219=DIRECTION('center_axis',(-0.707106781186549,0.,-0.707106781186546));
#13220=DIRECTION('ref_axis',(0.707106781186546,0.,-0.707106781186549));
#13221=DIRECTION('',(-1.,0.,0.));
#13222=DIRECTION('center_axis',(0.707106781186549,0.,-0.707106781186546));
#13223=DIRECTION('ref_axis',(-0.707106781186546,0.,-0.707106781186549));
#13224=DIRECTION('center_axis',(0.707106781186549,0.,0.707106781186546));
#13225=DIRECTION('ref_axis',(0.707106781186546,0.,-0.707106781186549));
#13226=DIRECTION('center_axis',(0.707106781186549,0.,-0.707106781186546));
#13227=DIRECTION('ref_axis',(-0.707106781186546,0.,-0.707106781186549));
#13228=DIRECTION('',(1.,0.,0.));
#13229=DIRECTION('center_axis',(-0.707106781186549,0.,-0.707106781186546));
#13230=DIRECTION('ref_axis',(0.707106781186546,0.,-0.707106781186549));
#13231=DIRECTION('center_axis',(-0.707106781186549,0.,0.707106781186546));
#13232=DIRECTION('ref_axis',(-0.707106781186546,0.,-0.707106781186549));
#13233=DIRECTION('center_axis',(0.,0.,1.));
#13234=DIRECTION('ref_axis',(1.,0.,0.));
#13235=DIRECTION('center_axis',(0.,0.,1.));
#13236=DIRECTION('ref_axis',(1.,0.,0.));
#13237=DIRECTION('center_axis',(0.,0.,1.));
#13238=DIRECTION('ref_axis',(1.,0.,0.));
#13239=DIRECTION('center_axis',(0.,0.,1.));
#13240=DIRECTION('ref_axis',(1.,0.,0.));
#13241=DIRECTION('center_axis',(0.,0.,1.));
#13242=DIRECTION('ref_axis',(1.,0.,0.));
#13243=DIRECTION('center_axis',(0.,0.,1.));
#13244=DIRECTION('ref_axis',(1.,0.,0.));
#13245=DIRECTION('center_axis',(0.,0.,1.));
#13246=DIRECTION('ref_axis',(1.,0.,0.));
#13247=DIRECTION('center_axis',(0.,0.,1.));
#13248=DIRECTION('ref_axis',(1.,0.,0.));
#13249=DIRECTION('',(0.,0.,1.));
#13250=DIRECTION('center_axis',(1.,0.,0.));
#13251=DIRECTION('ref_axis',(0.,1.,0.));
#13252=DIRECTION('',(0.,1.,0.));
#13253=DIRECTION('center_axis',(-1.,0.,0.));
#13254=DIRECTION('ref_axis',(0.,-1.,0.));
#13255=DIRECTION('',(0.,-1.,0.));
#13256=DIRECTION('center_axis',(0.,0.,1.));
#13257=DIRECTION('ref_axis',(1.,0.,0.));
#16382=CARTESIAN_POINT('',(0.,0.,0.));
#16383=CARTESIAN_POINT('Origin',(0.7,10.7,7.6));
#16384=CARTESIAN_POINT('',(0.96457513110646,10.4,7.6));
#16385=CARTESIAN_POINT('',(0.435424868893539,10.4,7.6));
#16386=CARTESIAN_POINT('',(-0.9,10.4,7.6));
#16387=CARTESIAN_POINT('Origin',(0.7,10.7,7.6));
#16388=CARTESIAN_POINT('',(0.475,10.7,7.6));
#16389=CARTESIAN_POINT('Origin',(0.7,10.7,7.6));
#16390=CARTESIAN_POINT('Origin',(0.7,10.7,7.6));
#16391=CARTESIAN_POINT('',(0.96457513110646,10.4,10.));
#16392=CARTESIAN_POINT('',(0.96457513110646,10.4,7.6));
#16393=CARTESIAN_POINT('',(0.435424868893539,10.4,10.));
#16394=CARTESIAN_POINT('Origin',(0.7,10.7,10.));
#16395=CARTESIAN_POINT('',(0.435424868893539,10.4,7.6));
#16396=CARTESIAN_POINT('Origin',(-0.7,12.1,7.6));
#16397=CARTESIAN_POINT('',(-0.964575131106458,12.4,7.6));
#16398=CARTESIAN_POINT('',(-0.435424868893542,12.4,7.6));
#16399=CARTESIAN_POINT('',(0.9,12.4,7.6));
#16400=CARTESIAN_POINT('Origin',(-0.7,12.1,7.6));
#16401=CARTESIAN_POINT('',(-0.925,12.1,7.6));
#16402=CARTESIAN_POINT('Origin',(-0.7,12.1,7.6));
#16403=CARTESIAN_POINT('Origin',(-0.7,12.1,7.6));
#16404=CARTESIAN_POINT('',(-0.964575131106458,12.4,10.));
#16405=CARTESIAN_POINT('',(-0.964575131106458,12.4,7.6));
#16406=CARTESIAN_POINT('',(-0.435424868893542,12.4,10.));
#16407=CARTESIAN_POINT('Origin',(-0.7,12.1,10.));
#16408=CARTESIAN_POINT('',(-0.435424868893542,12.4,7.6));
#16409=CARTESIAN_POINT('Origin',(-0.7,10.7,7.6));
#16410=CARTESIAN_POINT('',(-0.43542486889354,10.4,7.6));
#16411=CARTESIAN_POINT('',(-0.96457513110646,10.4,7.6));
#16412=CARTESIAN_POINT('',(-1.6,10.4,7.6));
#16413=CARTESIAN_POINT('Origin',(-0.7,10.7,7.6));
#16414=CARTESIAN_POINT('',(-0.925,10.7,7.6));
#16415=CARTESIAN_POINT('Origin',(-0.7,10.7,7.6));
#16416=CARTESIAN_POINT('Origin',(-0.7,10.7,7.6));
#16417=CARTESIAN_POINT('',(-0.43542486889354,10.4,10.));
#16418=CARTESIAN_POINT('',(-0.43542486889354,10.4,7.6));
#16419=CARTESIAN_POINT('',(-0.96457513110646,10.4,10.));
#16420=CARTESIAN_POINT('Origin',(-0.7,10.7,10.));
#16421=CARTESIAN_POINT('',(-0.96457513110646,10.4,7.6));
#16422=CARTESIAN_POINT('Origin',(0.7,12.1,7.6));
#16423=CARTESIAN_POINT('',(0.435424868893541,12.4,7.6));
#16424=CARTESIAN_POINT('',(0.964575131106458,12.4,7.6));
#16425=CARTESIAN_POINT('',(1.6,12.4,7.6));
#16426=CARTESIAN_POINT('Origin',(0.7,12.1,7.6));
#16427=CARTESIAN_POINT('',(0.475,12.1,7.6));
#16428=CARTESIAN_POINT('Origin',(0.7,12.1,7.6));
#16429=CARTESIAN_POINT('Origin',(0.7,12.1,7.6));
#16430=CARTESIAN_POINT('',(0.435424868893541,12.4,10.));
#16431=CARTESIAN_POINT('',(0.435424868893541,12.4,7.6));
#16432=CARTESIAN_POINT('',(0.964575131106458,12.4,10.));
#16433=CARTESIAN_POINT('Origin',(0.7,12.1,10.));
#16434=CARTESIAN_POINT('',(0.964575131106458,12.4,7.6));
#16435=CARTESIAN_POINT('Origin',(-2.5,10.4,7.));
#16436=CARTESIAN_POINT('',(-2.5,10.4,10.));
#16437=CARTESIAN_POINT('',(-2.5,10.4,10.));
#16438=CARTESIAN_POINT('',(-2.5,10.4,10.));
#16439=CARTESIAN_POINT('',(-2.5,10.4,7.));
#16440=CARTESIAN_POINT('',(-2.5,10.4,7.));
#16441=CARTESIAN_POINT('',(2.5,10.4,7.));
#16442=CARTESIAN_POINT('',(-2.5,10.4,7.));
#16443=CARTESIAN_POINT('',(2.5,10.4,10.));
#16444=CARTESIAN_POINT('',(2.5,10.4,7.));
#16445=CARTESIAN_POINT('',(-2.5,10.4,10.));
#16446=CARTESIAN_POINT('Origin',(0.,11.4,10.));
#16447=CARTESIAN_POINT('',(2.5,12.4,10.));
#16448=CARTESIAN_POINT('',(2.5,10.4,10.));
#16449=CARTESIAN_POINT('',(2.5,12.4,10.));
#16450=CARTESIAN_POINT('',(2.5,12.4,10.));
#16451=CARTESIAN_POINT('',(-2.5,12.4,10.));
#16452=CARTESIAN_POINT('',(2.5,12.4,10.));
#16453=CARTESIAN_POINT('',(-2.5,12.4,10.));
#16454=CARTESIAN_POINT('',(0.985,11.4,10.));
#16455=CARTESIAN_POINT('Origin',(1.5,11.4,10.));
#16456=CARTESIAN_POINT('',(-2.015,11.4,10.));
#16457=CARTESIAN_POINT('Origin',(-1.5,11.4,10.));
#16458=CARTESIAN_POINT('Origin',(2.5,12.4,7.));
#16459=CARTESIAN_POINT('',(2.5,12.4,7.));
#16460=CARTESIAN_POINT('',(2.5,12.4,7.));
#16461=CARTESIAN_POINT('',(-2.5,12.4,7.));
#16462=CARTESIAN_POINT('',(2.5,12.4,7.));
#16463=CARTESIAN_POINT('',(-2.5,12.4,7.));
#16464=CARTESIAN_POINT('Origin',(0.7,10.7,6.9));
#16465=CARTESIAN_POINT('',(0.475,10.7,7.));
#16466=CARTESIAN_POINT('Origin',(0.7,10.7,7.));
#16467=CARTESIAN_POINT('',(0.475,10.7,6.9));
#16468=CARTESIAN_POINT('Origin',(-0.7,12.1,6.9));
#16469=CARTESIAN_POINT('',(-0.925,12.1,7.));
#16470=CARTESIAN_POINT('Origin',(-0.7,12.1,7.));
#16471=CARTESIAN_POINT('',(-0.925,12.1,6.9));
#16472=CARTESIAN_POINT('Origin',(-0.7,10.7,6.9));
#16473=CARTESIAN_POINT('',(-0.925,10.7,7.));
#16474=CARTESIAN_POINT('Origin',(-0.7,10.7,7.));
#16475=CARTESIAN_POINT('',(-0.925,10.7,6.9));
#16476=CARTESIAN_POINT('Origin',(0.7,12.1,6.9));
#16477=CARTESIAN_POINT('',(0.475,12.1,7.));
#16478=CARTESIAN_POINT('Origin',(0.7,12.1,7.));
#16479=CARTESIAN_POINT('',(0.475,12.1,6.9));
#16480=CARTESIAN_POINT('Origin',(1.5,11.4,9.35));
#16481=CARTESIAN_POINT('',(0.985,11.4,9.35));
#16482=CARTESIAN_POINT('Origin',(1.5,11.4,9.35));
#16483=CARTESIAN_POINT('',(0.985,11.4,9.35));
#16484=CARTESIAN_POINT('Origin',(1.5,11.4,9.35));
#16485=CARTESIAN_POINT('',(1.1,11.4,9.35));
#16486=CARTESIAN_POINT('Origin',(1.5,11.4,9.35));
#16487=CARTESIAN_POINT('Origin',(1.5,11.4,8.42));
#16488=CARTESIAN_POINT('',(1.1,11.4,8.42));
#16489=CARTESIAN_POINT('Origin',(1.5,11.4,8.42));
#16490=CARTESIAN_POINT('',(1.1,11.4,8.42));
#16491=CARTESIAN_POINT('Origin',(1.5,11.4,8.42));
#16492=CARTESIAN_POINT('',(1.26,11.4,8.42));
#16493=CARTESIAN_POINT('Origin',(1.5,11.4,8.42));
#16494=CARTESIAN_POINT('Origin',(1.5,11.4,8.2));
#16495=CARTESIAN_POINT('',(1.26,11.4,8.3));
#16496=CARTESIAN_POINT('Origin',(1.5,11.4,8.3));
#16497=CARTESIAN_POINT('',(1.26,11.4,8.2));
#16498=CARTESIAN_POINT('Origin',(1.5,11.4,8.));
#16499=CARTESIAN_POINT('',(1.1394448724536,11.2267949192431,8.));
#16500=CARTESIAN_POINT('',(1.5,11.2267949192431,8.));
#16501=CARTESIAN_POINT('',(-1.5,11.2267949192431,8.));
#16502=CARTESIAN_POINT('',(1.1394448724536,11.5732050807569,8.));
#16503=CARTESIAN_POINT('Origin',(1.5,11.4,8.));
#16504=CARTESIAN_POINT('',(1.5,11.5732050807569,8.));
#16505=CARTESIAN_POINT('',(-1.5,11.5732050807569,8.));
#16506=CARTESIAN_POINT('',(1.5,11.4,8.));
#16507=CARTESIAN_POINT('Origin',(1.5,11.4,8.));
#16508=CARTESIAN_POINT('',(1.1,11.4,8.3));
#16509=CARTESIAN_POINT('Ctrl Pts',(1.1,11.4,8.3));
#16510=CARTESIAN_POINT('Ctrl Pts',(1.1,11.3744089397783,8.3));
#16511=CARTESIAN_POINT('Ctrl Pts',(1.10268160632987,11.3474109849022,8.29479278117383));
#16512=CARTESIAN_POINT('Ctrl Pts',(1.1123470317921,11.2982518483771,8.27423301598492));
#16513=CARTESIAN_POINT('Ctrl Pts',(1.1192266779859,11.2760606660387,8.25890337851337));
#16514=CARTESIAN_POINT('Ctrl Pts',(1.13245990649023,11.2410488343738,8.22389154684841));
#16515=CARTESIAN_POINT('Ctrl Pts',(1.13976079750786,11.2257542580528,8.20171647190156));
#16516=CARTESIAN_POINT('Ctrl Pts',(1.15043491280941,11.2052228831046,8.15262772025265));
#16517=CARTESIAN_POINT('Ctrl Pts',(1.15358983848623,11.2,8.1256610133921));
#16518=CARTESIAN_POINT('Ctrl Pts',(1.15358983848623,11.2,8.0743389866079));
#16519=CARTESIAN_POINT('Ctrl Pts',(1.15043491280941,11.2052228831046,8.04737227974735));
#16520=CARTESIAN_POINT('Ctrl Pts',(1.14338612646599,11.2187810348819,8.0149559049506));
#16521=CARTESIAN_POINT('Ctrl Pts',(1.14147391087861,11.2225711389422,8.00731580208126));
#16522=CARTESIAN_POINT('Ctrl Pts',(1.1394448724536,11.2267949192431,8.));
#16523=CARTESIAN_POINT('Origin',(1.5,11.4,8.3));
#16524=CARTESIAN_POINT('Ctrl Pts',(1.1394448724536,11.5732050807569,8.));
#16525=CARTESIAN_POINT('Ctrl Pts',(1.14147391087861,11.5774288610578,8.00731580208126));
#16526=CARTESIAN_POINT('Ctrl Pts',(1.14338612646599,11.5812189651181,8.01495590495059));
#16527=CARTESIAN_POINT('Ctrl Pts',(1.15043491280941,11.5947771168954,8.04737227974734));
#16528=CARTESIAN_POINT('Ctrl Pts',(1.15358983848623,11.6,8.0743389866079));
#16529=CARTESIAN_POINT('Ctrl Pts',(1.15358983848623,11.6,8.1));
#16530=CARTESIAN_POINT('Ctrl Pts',(1.15358983848623,11.6,8.1256610133921));
#16531=CARTESIAN_POINT('Ctrl Pts',(1.15043491280941,11.5947771168954,8.15262772025265));
#16532=CARTESIAN_POINT('Ctrl Pts',(1.13976079750786,11.5742457419472,8.20171647190156));
#16533=CARTESIAN_POINT('Ctrl Pts',(1.13245990649023,11.5589511656262,8.22389154684841));
#16534=CARTESIAN_POINT('Ctrl Pts',(1.1192266779859,11.5239393339613,8.25890337851337));
#16535=CARTESIAN_POINT('Ctrl Pts',(1.1123470317921,11.5017481516229,8.27423301598492));
#16536=CARTESIAN_POINT('Ctrl Pts',(1.10268160632987,11.4525890150978,8.29479278117383));
#16537=CARTESIAN_POINT('Ctrl Pts',(1.1,11.4255910602217,8.3));
#16538=CARTESIAN_POINT('Ctrl Pts',(1.1,11.4,8.3));
#16539=CARTESIAN_POINT('Origin',(1.5,11.4,8.3));
#16540=CARTESIAN_POINT('Origin',(1.5,11.4,8.1));
#16541=CARTESIAN_POINT('Origin',(1.5,11.4,8.1));
#16542=CARTESIAN_POINT('Origin',(-1.5,11.4,9.35));
#16543=CARTESIAN_POINT('',(-2.015,11.4,9.35));
#16544=CARTESIAN_POINT('Origin',(-1.5,11.4,9.35));
#16545=CARTESIAN_POINT('',(-2.015,11.4,9.35));
#16546=CARTESIAN_POINT('Origin',(-1.5,11.4,9.35));
#16547=CARTESIAN_POINT('',(-1.9,11.4,9.35));
#16548=CARTESIAN_POINT('Origin',(-1.5,11.4,9.35));
#16549=CARTESIAN_POINT('Origin',(-1.5,11.4,9.));
#16550=CARTESIAN_POINT('',(-1.9,11.4,9.));
#16551=CARTESIAN_POINT('Origin',(-1.5,11.4,9.));
#16552=CARTESIAN_POINT('',(-1.9,11.4,9.));
#16553=CARTESIAN_POINT('Origin',(-1.5,11.4,9.));
#16554=CARTESIAN_POINT('',(-1.74,11.4,9.));
#16555=CARTESIAN_POINT('Origin',(-1.5,11.4,9.));
#16556=CARTESIAN_POINT('Origin',(-1.5,11.4,8.2));
#16557=CARTESIAN_POINT('',(-1.74,11.4,8.78));
#16558=CARTESIAN_POINT('Origin',(-1.5,11.4,8.78));
#16559=CARTESIAN_POINT('',(-1.74,11.4,8.2));
#16560=CARTESIAN_POINT('Origin',(-1.5,11.4,8.));
#16561=CARTESIAN_POINT('',(-1.1394448724536,11.5732050807569,8.));
#16562=CARTESIAN_POINT('',(-1.5,11.5732050807569,8.));
#16563=CARTESIAN_POINT('',(-1.5,11.5732050807569,8.));
#16564=CARTESIAN_POINT('',(-1.9,11.4,8.));
#16565=CARTESIAN_POINT('Origin',(-1.5,11.4,8.));
#16566=CARTESIAN_POINT('',(-1.1394448724536,11.2267949192431,8.));
#16567=CARTESIAN_POINT('Origin',(-1.5,11.4,8.));
#16568=CARTESIAN_POINT('',(-1.5,11.2267949192431,8.));
#16569=CARTESIAN_POINT('',(-1.5,11.2267949192431,8.));
#16570=CARTESIAN_POINT('',(-1.5,11.4,8.));
#16571=CARTESIAN_POINT('Origin',(-1.5,11.4,8.));
#16572=CARTESIAN_POINT('',(-1.1,11.4,8.3));
#16573=CARTESIAN_POINT('Ctrl Pts',(-1.1394448724536,11.2267949192431,8.));
#16574=CARTESIAN_POINT('Ctrl Pts',(-1.14147391087861,11.2225711389422,8.00731580208126));
#16575=CARTESIAN_POINT('Ctrl Pts',(-1.14338612646599,11.2187810348819,8.0149559049506));
#16576=CARTESIAN_POINT('Ctrl Pts',(-1.15043491280941,11.2052228831046,8.04737227974735));
#16577=CARTESIAN_POINT('Ctrl Pts',(-1.15358983848623,11.2,8.0743389866079));
#16578=CARTESIAN_POINT('Ctrl Pts',(-1.15358983848623,11.2,8.1256610133921));
#16579=CARTESIAN_POINT('Ctrl Pts',(-1.15043491280941,11.2052228831046,8.15262772025265));
#16580=CARTESIAN_POINT('Ctrl Pts',(-1.13976079750786,11.2257542580528,8.20171647190156));
#16581=CARTESIAN_POINT('Ctrl Pts',(-1.13245990649023,11.2410488343738,8.22389154684841));
#16582=CARTESIAN_POINT('Ctrl Pts',(-1.1192266779859,11.2760606660387,8.25890337851337));
#16583=CARTESIAN_POINT('Ctrl Pts',(-1.1123470317921,11.2982518483771,8.27423301598492));
#16584=CARTESIAN_POINT('Ctrl Pts',(-1.10268160632987,11.3474109849022,8.29479278117383));
#16585=CARTESIAN_POINT('Ctrl Pts',(-1.1,11.3744089397783,8.3));
#16586=CARTESIAN_POINT('Ctrl Pts',(-1.1,11.4,8.3));
#16587=CARTESIAN_POINT('',(-1.9,11.4,8.78));
#16588=CARTESIAN_POINT('',(-1.9,11.4,8.));
#16589=CARTESIAN_POINT('Origin',(-1.5,11.4,8.78));
#16590=CARTESIAN_POINT('Ctrl Pts',(-1.1,11.4,8.3));
#16591=CARTESIAN_POINT('Ctrl Pts',(-1.1,11.4255910602217,8.3));
#16592=CARTESIAN_POINT('Ctrl Pts',(-1.10268160632987,11.4525890150978,8.29479278117383));
#16593=CARTESIAN_POINT('Ctrl Pts',(-1.1123470317921,11.5017481516229,8.27423301598492));
#16594=CARTESIAN_POINT('Ctrl Pts',(-1.1192266779859,11.5239393339613,8.25890337851337));
#16595=CARTESIAN_POINT('Ctrl Pts',(-1.13245990649023,11.5589511656262,8.22389154684841));
#16596=CARTESIAN_POINT('Ctrl Pts',(-1.13976079750786,11.5742457419472,8.20171647190156));
#16597=CARTESIAN_POINT('Ctrl Pts',(-1.15043491280941,11.5947771168954,8.15262772025265));
#16598=CARTESIAN_POINT('Ctrl Pts',(-1.15358983848623,11.6,8.1256610133921));
#16599=CARTESIAN_POINT('Ctrl Pts',(-1.15358983848623,11.6,8.1));
#16600=CARTESIAN_POINT('Ctrl Pts',(-1.15358983848623,11.6,8.0743389866079));
#16601=CARTESIAN_POINT('Ctrl Pts',(-1.15043491280941,11.5947771168954,8.04737227974735));
#16602=CARTESIAN_POINT('Ctrl Pts',(-1.14338612646599,11.5812189651181,8.01495590495059));
#16603=CARTESIAN_POINT('Ctrl Pts',(-1.14147391087861,11.5774288610578,8.00731580208127));
#16604=CARTESIAN_POINT('Ctrl Pts',(-1.1394448724536,11.5732050807569,8.));
#16605=CARTESIAN_POINT('Origin',(-1.5,11.4,8.78));
#16606=CARTESIAN_POINT('Origin',(-1.5,11.4,8.1));
#16607=CARTESIAN_POINT('Origin',(-1.5,11.4,8.1));
#16608=CARTESIAN_POINT('Origin',(-1.5,11.4,8.1));
#16609=CARTESIAN_POINT('',(-1.5,11.4,8.3));
#16610=CARTESIAN_POINT('',(0.,11.6,8.1));
#16611=CARTESIAN_POINT('',(-0.199999999999999,11.4,7.9));
#16612=CARTESIAN_POINT('Origin',(0.,11.4,8.1));
#16613=CARTESIAN_POINT('',(-0.1,11.5732050807569,8.2));
#16614=CARTESIAN_POINT('Origin',(0.,11.4,8.1));
#16615=CARTESIAN_POINT('',(0.1,11.5732050807569,8.2));
#16616=CARTESIAN_POINT('',(-1.5,11.5732050807569,8.2));
#16617=CARTESIAN_POINT('Origin',(0.,11.4,8.1));
#16618=CARTESIAN_POINT('',(0.,11.2,8.1));
#16619=CARTESIAN_POINT('Origin',(0.,11.4,8.1));
#16620=CARTESIAN_POINT('',(0.1,11.2267949192431,8.2));
#16621=CARTESIAN_POINT('Origin',(0.,11.4,8.1));
#16622=CARTESIAN_POINT('',(-0.1,11.2267949192431,8.2));
#16623=CARTESIAN_POINT('',(-1.5,11.2267949192431,8.2));
#16624=CARTESIAN_POINT('Origin',(0.,11.4,8.1));
#16625=CARTESIAN_POINT('Origin',(0.,11.4,8.1));
#16626=CARTESIAN_POINT('Origin',(0.,11.4,8.2));
#16627=CARTESIAN_POINT('Origin',(0.,11.4,8.2));
#16628=CARTESIAN_POINT('Origin',(0.,11.4,8.2));
#16629=CARTESIAN_POINT('Origin',(0.,11.4,8.2));
#16630=CARTESIAN_POINT('Origin',(0.,11.4,6.9));
#16631=CARTESIAN_POINT('Origin',(0.,11.4,6.9));
#16632=CARTESIAN_POINT('Origin',(0.,11.4,6.9));
#16633=CARTESIAN_POINT('',(-0.2,11.4,7.));
#16634=CARTESIAN_POINT('Origin',(0.,11.4,7.));
#16635=CARTESIAN_POINT('',(-0.2,11.4,6.9));
#16636=CARTESIAN_POINT('Origin',(2.5,10.4,7.));
#16637=CARTESIAN_POINT('',(2.5,10.4,7.));
#16638=CARTESIAN_POINT('Origin',(-2.5,12.4,7.));
#16639=CARTESIAN_POINT('',(-2.5,12.4,7.));
#16640=CARTESIAN_POINT('Origin',(0.,11.4,7.));
#18934=UNCERTAINTY_MEASURE_WITH_UNIT(LENGTH_MEASURE(0.001),#19044,
'DISTANCE_ACCURACY_VALUE',
'Maximum model space distance between geometric entities at asserted c
onnectivities');
#18972=UNCERTAINTY_MEASURE_WITH_UNIT(LENGTH_MEASURE(0.001),#19044,
'DISTANCE_ACCURACY_VALUE',
'Maximum model space distance between geometric entities at asserted c
onnectivities');
#19005=(
GEOMETRIC_REPRESENTATION_CONTEXT(3)
GLOBAL_UNCERTAINTY_ASSIGNED_CONTEXT((#18934))
GLOBAL_UNIT_ASSIGNED_CONTEXT((#19044,#19046,#19047))
REPRESENTATION_CONTEXT('','3D')
);
#19043=(
GEOMETRIC_REPRESENTATION_CONTEXT(3)
GLOBAL_UNCERTAINTY_ASSIGNED_CONTEXT((#18972))
GLOBAL_UNIT_ASSIGNED_CONTEXT((#19044,#19046,#19047))
REPRESENTATION_CONTEXT('','3D')
);
#19044=(
LENGTH_UNIT()
NAMED_UNIT(*)
SI_UNIT(.CENTI.,.METRE.)
);
#19046=(
NAMED_UNIT(*)
PLANE_ANGLE_UNIT()
SI_UNIT($,.RADIAN.)
);
#19047=(
NAMED_UNIT(*)
SI_UNIT($,.STERADIAN.)
SOLID_ANGLE_UNIT()
);
#19080=SHAPE_DEFINITION_REPRESENTATION(#19155,#19338);
#19155=PRODUCT_DEFINITION_SHAPE('',$,#19409);
#19338=SHAPE_REPRESENTATION('',(#10863),#19005);
#19376=PRODUCT_DEFINITION_CONTEXT('part definition',#19588,'design');
#19409=PRODUCT_DEFINITION('2026-11-03-00-38-46-488',
'Check valve manifold',#19479,#19376);
#19479=PRODUCT_DEFINITION_FORMATION('',$,#19622);
#19588=APPLICATION_CONTEXT(
'Core Data for Automotive Mechanical Design Process');
#19589=PRODUCT_CONTEXT('part definition',#19588,'mechanical');
#19622=PRODUCT('2026-11-03-00-38-46-488','Check valve manifold',
'Check valve manifold',(#19589));
#19661=PRESENTATION_STYLE_ASSIGNMENT((#19667));
#19667=SURFACE_STYLE_USAGE(.BOTH.,#19673);
#19673=SURFACE_SIDE_STYLE('',(#19679));
#19679=SURFACE_STYLE_FILL_AREA(#19685);
#19685=FILL_AREA_STYLE('CAD Library Painted - Engineering blue',(#19691));
#19691=FILL_AREA_STYLE_COLOUR('CAD Library Painted - Engineering blue',
#19697);
#19697=COLOUR_RGB('CAD Library Painted - Engineering blue',0.12156862745098,
0.356862745098039,0.6);
ENDSEC;
END-ISO-10303-21;
